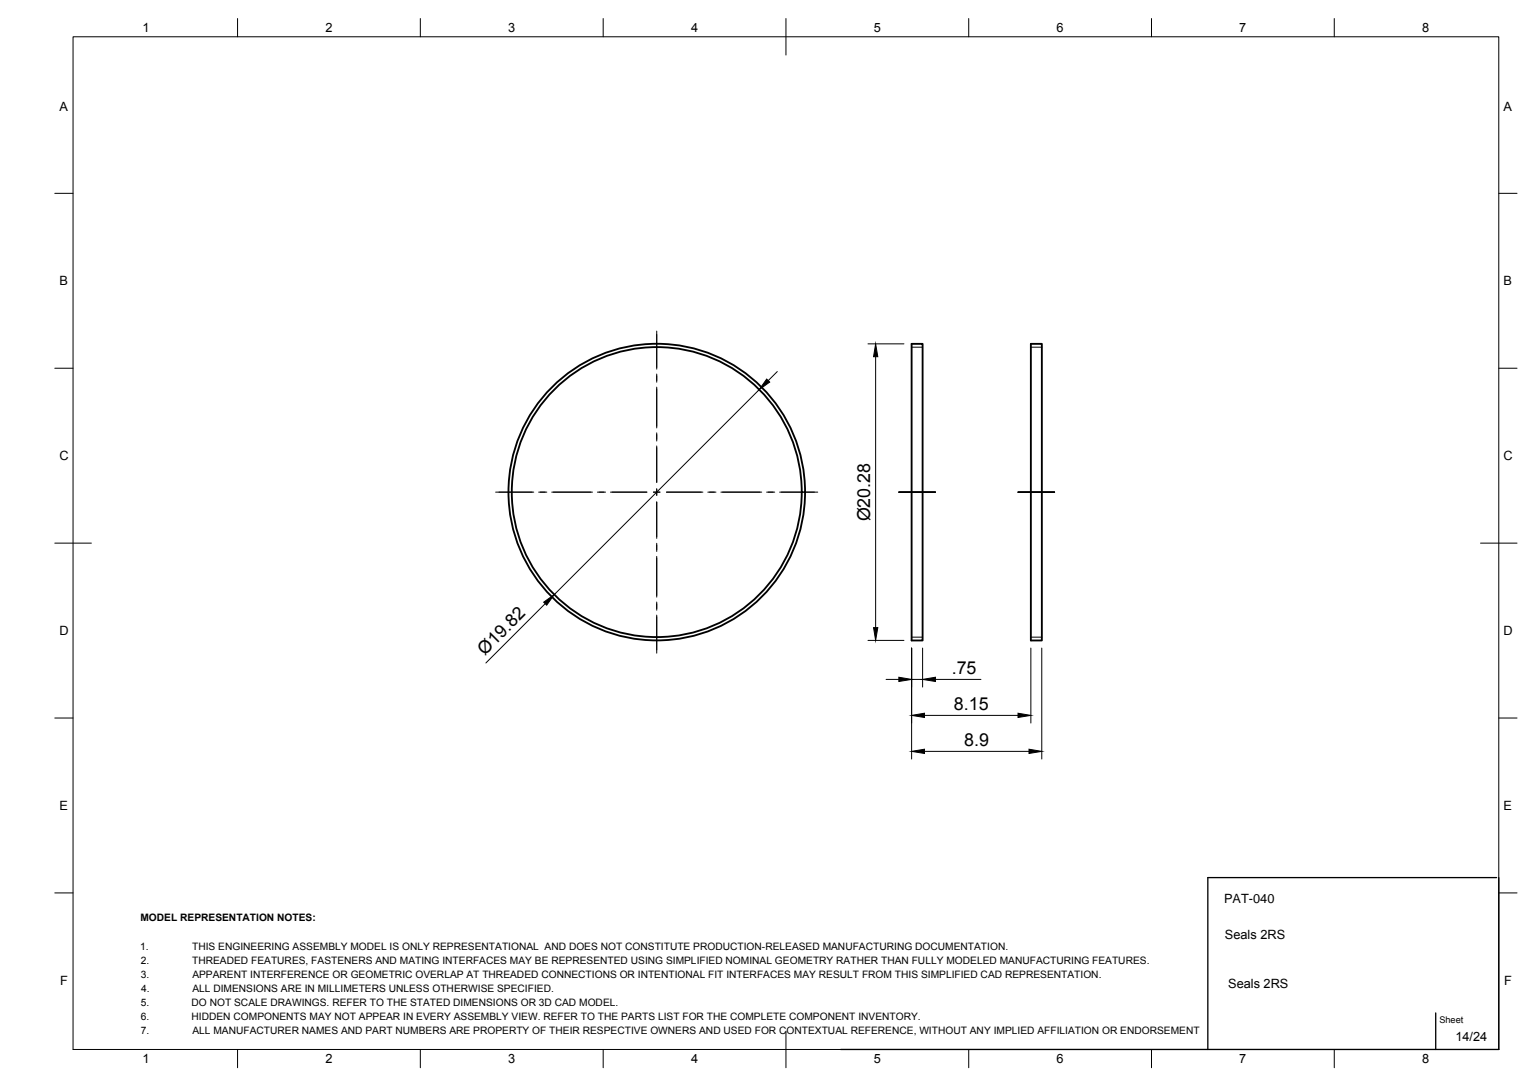
ISO-10303-21;
HEADER;
/* Generated by software containing ST-Developer
 * from STEP Tools, Inc. (www.steptools.com) 
 */

FILE_DESCRIPTION(
/* description */ ('Four-bar tabletop demonstrator'),
/* implementation_level */ '2;1');

FILE_NAME(
/* name */ 'Seals 2RS.step',
/* time_stamp */ '2026-10-29T17:05:23-07:00',
/* author */ (''),
/* organization */ (''),
/* preprocessor_version */ 'ST-DEVELOPER v20.2',
/* originating_system */ 'Autodesk Translation Framework v15.17.0.0',
/* authorisation */ '');

FILE_SCHEMA (('AUTOMOTIVE_DESIGN { 1 0 10303 214 3 1 1 }'));
ENDSEC;

DATA;
#10=MECHANICAL_DESIGN_GEOMETRIC_PRESENTATION_REPRESENTATION('',(#352,#353),#6705);
#315=SHAPE_REPRESENTATION_RELATIONSHIP('SRR','None',#6824,#330);
#330=ADVANCED_BREP_SHAPE_REPRESENTATION('',(#374,#375),#6697);
#352=STYLED_ITEM('',(#6989),#374);
#353=STYLED_ITEM('',(#6989),#375);
#374=MANIFOLD_SOLID_BREP('Body1',#3397);
#375=MANIFOLD_SOLID_BREP('Body2',#3398);
#431=FACE_BOUND('',#941,.T.);
#432=FACE_BOUND('',#944,.T.);
#433=FACE_BOUND('',#947,.T.);
#434=FACE_BOUND('',#950,.T.);
#517=PLANE('',#3860);
#518=PLANE('',#3865);
#519=PLANE('',#3868);
#520=PLANE('',#3873);
#687=FACE_OUTER_BOUND('',#940,.T.);
#688=FACE_OUTER_BOUND('',#942,.T.);
#689=FACE_OUTER_BOUND('',#943,.T.);
#690=FACE_OUTER_BOUND('',#945,.T.);
#691=FACE_OUTER_BOUND('',#946,.T.);
#692=FACE_OUTER_BOUND('',#948,.T.);
#693=FACE_OUTER_BOUND('',#949,.T.);
#694=FACE_OUTER_BOUND('',#951,.T.);
#940=EDGE_LOOP('',(#2816));
#941=EDGE_LOOP('',(#2817));
#942=EDGE_LOOP('',(#2818,#2819,#2820,#2821));
#943=EDGE_LOOP('',(#2822));
#944=EDGE_LOOP('',(#2823));
#945=EDGE_LOOP('',(#2824,#2825,#2826,#2827));
#946=EDGE_LOOP('',(#2828));
#947=EDGE_LOOP('',(#2829));
#948=EDGE_LOOP('',(#2830,#2831,#2832,#2833));
#949=EDGE_LOOP('',(#2834));
#950=EDGE_LOOP('',(#2835));
#951=EDGE_LOOP('',(#2836,#2837,#2838,#2839));
#1142=LINE('',#6226,#1312);
#1143=LINE('',#6231,#1313);
#1144=LINE('',#6240,#1314);
#1145=LINE('',#6245,#1315);
#1312=VECTOR('',#4745,1.013815);
#1313=VECTOR('',#4752,0.991185);
#1314=VECTOR('',#4763,1.013815);
#1315=VECTOR('',#4770,0.991185);
#1538=CIRCLE('',#3861,1.013815);
#1539=CIRCLE('',#3862,0.991185);
#1540=CIRCLE('',#3864,1.013815);
#1541=CIRCLE('',#3866,0.991185);
#1542=CIRCLE('',#3869,1.013815);
#1543=CIRCLE('',#3870,0.991185);
#1544=CIRCLE('',#3872,1.013815);
#1545=CIRCLE('',#3874,0.991185);
#1785=VERTEX_POINT('',#6219);
#1786=VERTEX_POINT('',#6221);
#1787=VERTEX_POINT('',#6224);
#1788=VERTEX_POINT('',#6228);
#1789=VERTEX_POINT('',#6233);
#1790=VERTEX_POINT('',#6235);
#1791=VERTEX_POINT('',#6238);
#1792=VERTEX_POINT('',#6242);
#2144=EDGE_CURVE('',#1785,#1785,#1538,.T.);
#2145=EDGE_CURVE('',#1786,#1786,#1539,.T.);
#2146=EDGE_CURVE('',#1787,#1787,#1540,.T.);
#2147=EDGE_CURVE('',#1787,#1785,#1142,.T.);
#2148=EDGE_CURVE('',#1788,#1788,#1541,.T.);
#2149=EDGE_CURVE('',#1788,#1786,#1143,.T.);
#2150=EDGE_CURVE('',#1789,#1789,#1542,.T.);
#2151=EDGE_CURVE('',#1790,#1790,#1543,.T.);
#2152=EDGE_CURVE('',#1791,#1791,#1544,.T.);
#2153=EDGE_CURVE('',#1791,#1789,#1144,.T.);
#2154=EDGE_CURVE('',#1792,#1792,#1545,.T.);
#2155=EDGE_CURVE('',#1792,#1790,#1145,.T.);
#2816=ORIENTED_EDGE('',*,*,#2144,.F.);
#2817=ORIENTED_EDGE('',*,*,#2145,.T.);
#2818=ORIENTED_EDGE('',*,*,#2146,.F.);
#2819=ORIENTED_EDGE('',*,*,#2147,.T.);
#2820=ORIENTED_EDGE('',*,*,#2144,.T.);
#2821=ORIENTED_EDGE('',*,*,#2147,.F.);
#2822=ORIENTED_EDGE('',*,*,#2146,.T.);
#2823=ORIENTED_EDGE('',*,*,#2148,.F.);
#2824=ORIENTED_EDGE('',*,*,#2148,.T.);
#2825=ORIENTED_EDGE('',*,*,#2149,.T.);
#2826=ORIENTED_EDGE('',*,*,#2145,.F.);
#2827=ORIENTED_EDGE('',*,*,#2149,.F.);
#2828=ORIENTED_EDGE('',*,*,#2150,.F.);
#2829=ORIENTED_EDGE('',*,*,#2151,.T.);
#2830=ORIENTED_EDGE('',*,*,#2152,.F.);
#2831=ORIENTED_EDGE('',*,*,#2153,.T.);
#2832=ORIENTED_EDGE('',*,*,#2150,.T.);
#2833=ORIENTED_EDGE('',*,*,#2153,.F.);
#2834=ORIENTED_EDGE('',*,*,#2152,.T.);
#2835=ORIENTED_EDGE('',*,*,#2154,.F.);
#2836=ORIENTED_EDGE('',*,*,#2154,.T.);
#2837=ORIENTED_EDGE('',*,*,#2155,.T.);
#2838=ORIENTED_EDGE('',*,*,#2151,.F.);
#2839=ORIENTED_EDGE('',*,*,#2155,.F.);
#3149=CYLINDRICAL_SURFACE('',#3863,1.013815);
#3150=CYLINDRICAL_SURFACE('',#3867,0.991185);
#3151=CYLINDRICAL_SURFACE('',#3871,1.013815);
#3152=CYLINDRICAL_SURFACE('',#3875,0.991185);
#3303=ADVANCED_FACE('',(#687,#431),#517,.T.);
#3304=ADVANCED_FACE('',(#688),#3149,.T.);
#3305=ADVANCED_FACE('',(#689,#432),#518,.T.);
#3306=ADVANCED_FACE('',(#690),#3150,.F.);
#3307=ADVANCED_FACE('',(#691,#433),#519,.T.);
#3308=ADVANCED_FACE('',(#692),#3151,.T.);
#3309=ADVANCED_FACE('',(#693,#434),#520,.T.);
#3310=ADVANCED_FACE('',(#694),#3152,.F.);
#3397=CLOSED_SHELL('',(#3303,#3304,#3305,#3306));
#3398=CLOSED_SHELL('',(#3307,#3308,#3309,#3310));
#3859=AXIS2_PLACEMENT_3D('',#6217,#4733,#4734);
#3860=AXIS2_PLACEMENT_3D('',#6218,#4735,#4736);
#3861=AXIS2_PLACEMENT_3D('',#6220,#4737,#4738);
#3862=AXIS2_PLACEMENT_3D('',#6222,#4739,#4740);
#3863=AXIS2_PLACEMENT_3D('',#6223,#4741,#4742);
#3864=AXIS2_PLACEMENT_3D('',#6225,#4743,#4744);
#3865=AXIS2_PLACEMENT_3D('',#6227,#4746,#4747);
#3866=AXIS2_PLACEMENT_3D('',#6229,#4748,#4749);
#3867=AXIS2_PLACEMENT_3D('',#6230,#4750,#4751);
#3868=AXIS2_PLACEMENT_3D('',#6232,#4753,#4754);
#3869=AXIS2_PLACEMENT_3D('',#6234,#4755,#4756);
#3870=AXIS2_PLACEMENT_3D('',#6236,#4757,#4758);
#3871=AXIS2_PLACEMENT_3D('',#6237,#4759,#4760);
#3872=AXIS2_PLACEMENT_3D('',#6239,#4761,#4762);
#3873=AXIS2_PLACEMENT_3D('',#6241,#4764,#4765);
#3874=AXIS2_PLACEMENT_3D('',#6243,#4766,#4767);
#3875=AXIS2_PLACEMENT_3D('',#6244,#4768,#4769);
#4733=DIRECTION('axis',(0.,0.,1.));
#4734=DIRECTION('refdir',(1.,0.,0.));
#4735=DIRECTION('center_axis',(0.,1.,0.));
#4736=DIRECTION('ref_axis',(0.,0.,1.));
#4737=DIRECTION('center_axis',(0.,-1.,0.));
#4738=DIRECTION('ref_axis',(1.,0.,0.));
#4739=DIRECTION('center_axis',(0.,-1.,0.));
#4740=DIRECTION('ref_axis',(1.,0.,0.));
#4741=DIRECTION('center_axis',(0.,-1.,0.));
#4742=DIRECTION('ref_axis',(1.,0.,0.));
#4743=DIRECTION('center_axis',(0.,-1.,0.));
#4744=DIRECTION('ref_axis',(1.,0.,0.));
#4745=DIRECTION('',(0.,1.,0.));
#4746=DIRECTION('center_axis',(0.,-1.,0.));
#4747=DIRECTION('ref_axis',(0.,0.,-1.));
#4748=DIRECTION('center_axis',(0.,-1.,0.));
#4749=DIRECTION('ref_axis',(1.,0.,0.));
#4750=DIRECTION('center_axis',(0.,-1.,0.));
#4751=DIRECTION('ref_axis',(1.,0.,0.));
#4752=DIRECTION('',(0.,1.,0.));
#4753=DIRECTION('center_axis',(0.,1.,0.));
#4754=DIRECTION('ref_axis',(0.,0.,1.));
#4755=DIRECTION('center_axis',(0.,-1.,0.));
#4756=DIRECTION('ref_axis',(1.,0.,0.));
#4757=DIRECTION('center_axis',(0.,-1.,0.));
#4758=DIRECTION('ref_axis',(1.,0.,0.));
#4759=DIRECTION('center_axis',(0.,-1.,0.));
#4760=DIRECTION('ref_axis',(1.,0.,0.));
#4761=DIRECTION('center_axis',(0.,-1.,0.));
#4762=DIRECTION('ref_axis',(1.,0.,0.));
#4763=DIRECTION('',(0.,1.,0.));
#4764=DIRECTION('center_axis',(0.,-1.,0.));
#4765=DIRECTION('ref_axis',(0.,0.,-1.));
#4766=DIRECTION('center_axis',(0.,-1.,0.));
#4767=DIRECTION('ref_axis',(1.,0.,0.));
#4768=DIRECTION('center_axis',(0.,-1.,0.));
#4769=DIRECTION('ref_axis',(1.,0.,0.));
#4770=DIRECTION('',(0.,1.,0.));
#6217=CARTESIAN_POINT('',(0.,0.,0.));
#6218=CARTESIAN_POINT('Origin',(1.013815,0.445,0.));
#6219=CARTESIAN_POINT('',(-1.013815,0.445,-1.24156529467757E-16));
#6220=CARTESIAN_POINT('Origin',(0.,0.445,0.));
#6221=CARTESIAN_POINT('',(-0.991185,0.445,-1.21385153761287E-16));
#6222=CARTESIAN_POINT('Origin',(0.,0.445,0.));
#6223=CARTESIAN_POINT('Origin',(0.,0.4075,0.));
#6224=CARTESIAN_POINT('',(-1.013815,0.37,-1.24156529467757E-16));
#6225=CARTESIAN_POINT('Origin',(0.,0.37,0.));
#6226=CARTESIAN_POINT('',(-1.013815,0.4075,-1.24156529467757E-16));
#6227=CARTESIAN_POINT('Origin',(0.991185,0.37,0.));
#6228=CARTESIAN_POINT('',(-0.991185,0.37,-1.21385153761287E-16));
#6229=CARTESIAN_POINT('Origin',(0.,0.37,0.));
#6230=CARTESIAN_POINT('Origin',(0.,0.4075,0.));
#6231=CARTESIAN_POINT('',(-0.991185,0.4075,-1.21385153761287E-16));
#6232=CARTESIAN_POINT('Origin',(1.013815,-0.37,0.));
#6233=CARTESIAN_POINT('',(-1.013815,-0.37,-1.24156529467757E-16));
#6234=CARTESIAN_POINT('Origin',(0.,-0.37,0.));
#6235=CARTESIAN_POINT('',(-0.991185,-0.37,-1.21385153761287E-16));
#6236=CARTESIAN_POINT('Origin',(0.,-0.37,0.));
#6237=CARTESIAN_POINT('Origin',(0.,-0.4075,0.));
#6238=CARTESIAN_POINT('',(-1.013815,-0.445,-1.24156529467757E-16));
#6239=CARTESIAN_POINT('Origin',(0.,-0.445,0.));
#6240=CARTESIAN_POINT('',(-1.013815,-0.4075,-1.24156529467757E-16));
#6241=CARTESIAN_POINT('Origin',(0.991185,-0.445,0.));
#6242=CARTESIAN_POINT('',(-0.991185,-0.445,-1.21385153761287E-16));
#6243=CARTESIAN_POINT('Origin',(0.,-0.445,0.));
#6244=CARTESIAN_POINT('Origin',(0.,-0.4075,0.));
#6245=CARTESIAN_POINT('',(-0.991185,-0.4075,-1.21385153761287E-16));
#6675=UNCERTAINTY_MEASURE_WITH_UNIT(LENGTH_MEASURE(0.001),#6706,
'DISTANCE_ACCURACY_VALUE',
'Maximum model space distance between geometric entities at asserted c
onnectivities');
#6683=UNCERTAINTY_MEASURE_WITH_UNIT(LENGTH_MEASURE(0.001),#6706,
'DISTANCE_ACCURACY_VALUE',
'Maximum model space distance between geometric entities at asserted c
onnectivities');
#6697=(
GEOMETRIC_REPRESENTATION_CONTEXT(3)
GLOBAL_UNCERTAINTY_ASSIGNED_CONTEXT((#6675))
GLOBAL_UNIT_ASSIGNED_CONTEXT((#6706,#6708,#6709))
REPRESENTATION_CONTEXT('','3D')
);
#6705=(
GEOMETRIC_REPRESENTATION_CONTEXT(3)
GLOBAL_UNCERTAINTY_ASSIGNED_CONTEXT((#6683))
GLOBAL_UNIT_ASSIGNED_CONTEXT((#6706,#6708,#6709))
REPRESENTATION_CONTEXT('','3D')
);
#6706=(
LENGTH_UNIT()
NAMED_UNIT(*)
SI_UNIT(.CENTI.,.METRE.)
);
#6708=(
NAMED_UNIT(*)
PLANE_ANGLE_UNIT()
SI_UNIT($,.RADIAN.)
);
#6709=(
NAMED_UNIT(*)
SI_UNIT($,.STERADIAN.)
SOLID_ANGLE_UNIT()
);
#6723=SHAPE_DEFINITION_REPRESENTATION(#6744,#6824);
#6744=PRODUCT_DEFINITION_SHAPE('',$,#6846);
#6824=SHAPE_REPRESENTATION('',(#3859),#6697);
#6832=PRODUCT_DEFINITION_CONTEXT('part definition',#6897,'design');
#6846=PRODUCT_DEFINITION('Seals 2RS','Seals 2RS',#6867,#6832);
#6867=PRODUCT_DEFINITION_FORMATION('',$,#6912);
#6897=APPLICATION_CONTEXT(
'Core Data for Automotive Mechanical Design Process');
#6898=PRODUCT_CONTEXT('part definition',#6897,'mechanical');
#6912=PRODUCT('Seals 2RS','Seals 2RS','Seals 2RS',(#6898));
#6983=COLOUR_RGB('Grey',0.48,0.52,0.57);
#6984=FILL_AREA_STYLE_COLOUR('',#6983);
#6985=FILL_AREA_STYLE('',(#6984));
#6986=SURFACE_STYLE_FILL_AREA(#6985);
#6987=SURFACE_SIDE_STYLE('',(#6986));
#6988=SURFACE_STYLE_USAGE(.BOTH.,#6987);
#6989=PRESENTATION_STYLE_ASSIGNMENT((#6988));
ENDSEC;
END-ISO-10303-21;
